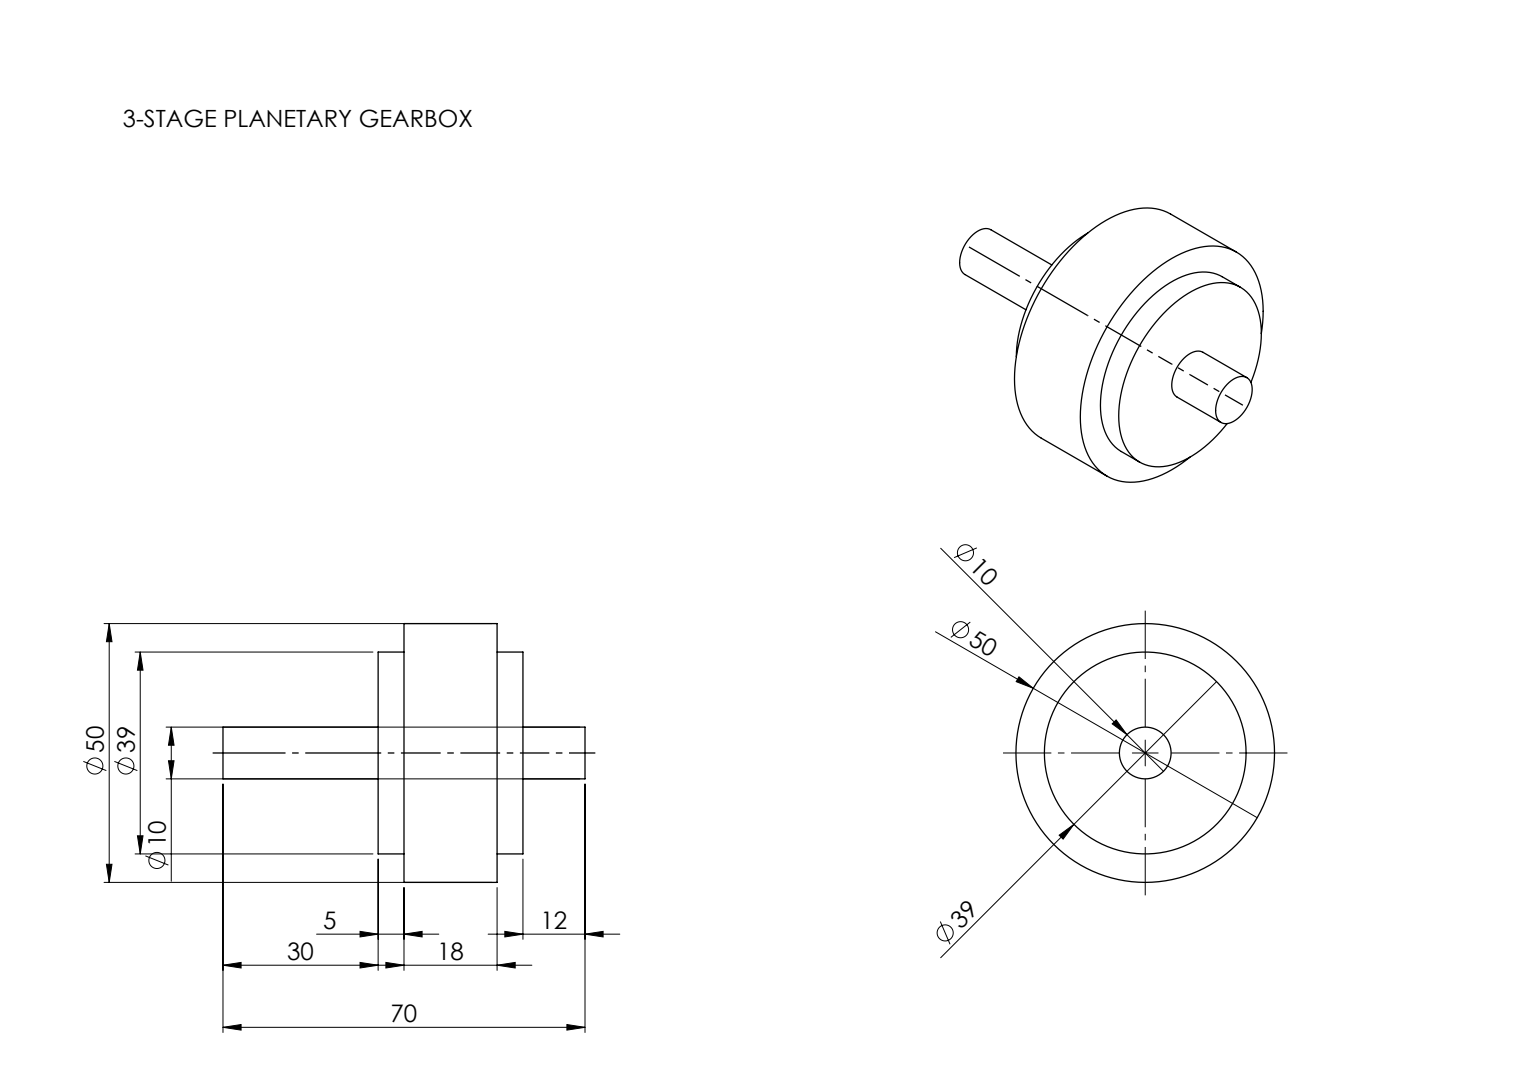
ISO-10303-21;
HEADER;
FILE_DESCRIPTION (('STEP AP214'),
    '1' );
FILE_NAME ('3-Stage Planetary Gearbox.step',
    '2026-10-05T20:22:16',
    ( '' ),
    ( '' ),
    'SwSTEP 2.0',
    'SolidWorks 2026',
    '' );
FILE_SCHEMA (( 'AUTOMOTIVE_DESIGN' ));
ENDSEC;

DATA;
#54=ORIENTED_EDGE ( 'NONE', *, *, #3388, .T. ) ;
#68=DIRECTION ( 'NONE',  ( 0.000000000000000000, 0.000000000000000000, 1.000000000000000000 ) ) ;
#87=DIRECTION ( 'NONE',  ( 0.000000000000000000, 0.000000000000000000, 1.000000000000000000 ) ) ;
#103=DIRECTION ( 'NONE',  ( 0.000000000000000000, 0.000000000000000000, 1.000000000000000000 ) ) ;
#119=ORIENTED_EDGE ( 'NONE', *, *, #7483, .T. ) ;
#126=ORIENTED_EDGE ( 'NONE', *, *, #14248, .F. ) ;
#235=EDGE_LOOP ( 'NONE', ( #13574, #321, #10866, #12718 ) ) ;
#261=CIRCLE ( 'NONE', #1953, 5.000000000000007994 ) ;
#301=CIRCLE ( 'NONE', #9619, 24.99999999999999645 ) ;
#313=VERTEX_POINT ( 'NONE', #2399 ) ;
#321=ORIENTED_EDGE ( 'NONE', *, *, #1465, .F. ) ;
#334=LINE ( 'NONE', #11212, #17228 ) ;
#345=EDGE_CURVE ( 'NONE', #10903, #313, #5234, .T. ) ;
#350=CARTESIAN_POINT ( 'NONE',  ( -50.00000000000000000, 171.6227766016838245, 24.99999999999999289 ) ) ;
#366=DIRECTION ( 'NONE',  ( -1.000000000000000000, -0.000000000000000000, -0.000000000000000000 ) ) ;
#432=AXIS2_PLACEMENT_3D ( 'NONE', #5586, #6655, #5500 ) ;
#446=EDGE_CURVE ( 'NONE', #9960, #12327, #12060, .T. ) ;
#485=CARTESIAN_POINT ( 'NONE',  ( -50.00000000000000000, 171.6227766016838245, 0.000000000000000000 ) ) ;
#508=DIRECTION ( 'NONE',  ( -1.000000000000000000, -0.000000000000000000, -0.000000000000000000 ) ) ;
#534=SURFACE_STYLE_USAGE ( .BOTH. , #5674 ) ;
#556=AXIS2_PLACEMENT_3D ( 'NONE', #15496, #7518, #2210 ) ;
#603=FACE_OUTER_BOUND ( 'NONE', #10174, .T. ) ;
#654=DIRECTION ( 'NONE',  ( -1.000000000000000000, 0.000000000000000000, 0.000000000000000000 ) ) ;
#713=VERTEX_POINT ( 'NONE', #3894 ) ;
#714=DIRECTION ( 'NONE',  ( 0.000000000000000000, 0.000000000000000000, -1.000000000000000000 ) ) ;
#771=FACE_BOUND ( 'NONE', #1719, .T. ) ;
#791=DIRECTION ( 'NONE',  ( -1.000000000000000000, 0.000000000000000000, 0.000000000000000000 ) ) ;
#836=CIRCLE ( 'NONE', #4239, 5.000000000000007994 ) ;
#866=AXIS2_PLACEMENT_3D ( 'NONE', #16436, #16167, #6863 ) ;
#886=ORIENTED_EDGE ( 'NONE', *, *, #9910, .T. ) ;
#990=CARTESIAN_POINT ( 'NONE',  ( -73.00000000000001421, 171.6227766016838245, 0.000000000000000000 ) ) ;
#1086=CARTESIAN_POINT ( 'NONE',  ( -73.00000000000001421, 171.6227766016838245, -5.000000000000007994 ) ) ;
#1147=CIRCLE ( 'NONE', #866, 24.99999999999999645 ) ;
#1200=DIRECTION ( 'NONE',  ( 0.000000000000000000, 0.000000000000000000, -1.000000000000000000 ) ) ;
#1235=FACE_OUTER_BOUND ( 'NONE', #1413, .T. ) ;
#1244=VECTOR ( 'NONE', #791, 1000.000000000000000 ) ;
#1354=DIRECTION ( 'NONE',  ( 0.000000000000000000, 0.000000000000000000, 1.000000000000000000 ) ) ;
#1360=ORIENTED_EDGE ( 'NONE', *, *, #6788, .T. ) ;
#1413=EDGE_LOOP ( 'NONE', ( #9423, #8176 ) ) ;
#1434=CIRCLE ( 'NONE', #13308, 5.000000000000007994 ) ;
#1465=EDGE_CURVE ( 'NONE', #10429, #16699, #5929, .T. ) ;
#1478=CARTESIAN_POINT ( 'NONE',  ( -33.00000000000000711, 171.6227766016838245, -5.000000000000007994 ) ) ;
#1490=CARTESIAN_POINT ( 'NONE',  ( -73.00000000000001421, 171.6227766016838245, 0.000000000000000000 ) ) ;
#1564=COLOUR_RGB ( '', 0.72549020, 0.75294118, 0.79215686) ;
#1569=CARTESIAN_POINT ( 'NONE',  ( -33.00000000000000711, 171.6227766016838245, 0.000000000000000000 ) ) ;
#1608=AXIS2_PLACEMENT_3D ( 'NONE', #16914, #3374, #714 ) ;
#1684=DIRECTION ( 'NONE',  ( -1.000000000000000000, 0.000000000000000000, 0.000000000000000000 ) ) ;
#1719=EDGE_LOOP ( 'NONE', ( #15688, #11199 ) ) ;
#1728=CARTESIAN_POINT ( 'NONE',  ( -33.00000000000000711, 171.6227766016838245, 0.000000000000000000 ) ) ;
#1778=ORIENTED_EDGE ( 'NONE', *, *, #14248, .T. ) ;
#1781=ORIENTED_EDGE ( 'NONE', *, *, #10186, .F. ) ;
#1805=DIRECTION ( 'NONE',  ( 0.000000000000000000, 0.000000000000000000, 1.000000000000000000 ) ) ;
#1843=PRESENTATION_STYLE_ASSIGNMENT (( #8568 ) ) ;
#1873=DIRECTION ( 'NONE',  ( -1.000000000000000000, 0.000000000000000000, 0.000000000000000000 ) ) ;
#1953=AXIS2_PLACEMENT_3D ( 'NONE', #16994, #6015, #10077 ) ;
#1978=DIRECTION ( 'NONE',  ( 1.000000000000000000, 0.000000000000000000, 0.000000000000000000 ) ) ;
#2008=CARTESIAN_POINT ( 'NONE',  ( -45.00000000000000711, 171.6227766016838245, -5.000000000000007994 ) ) ;
#2037=ORIENTED_EDGE ( 'NONE', *, *, #13494, .F. ) ;
#2046=UNCERTAINTY_MEASURE_WITH_UNIT (LENGTH_MEASURE( 1.000000000000000082E-05 ), #7499, 'distance_accuracy_value', 'NONE');
#2058=EDGE_LOOP ( 'NONE', ( #1778, #886 ) ) ;
#2072=ORIENTED_EDGE ( 'NONE', *, *, #8190, .F. ) ;
#2184=ORIENTED_EDGE ( 'NONE', *, *, #10068, .T. ) ;
#2188=FILL_AREA_STYLE ('',( #5926 ) ) ;
#2200=ADVANCED_FACE ( 'NONE', ( #13212 ), #4020, .T. ) ;
#2210=DIRECTION ( 'NONE',  ( 0.000000000000000000, 0.000000000000000000, -1.000000000000000000 ) ) ;
#2240=DIRECTION ( 'NONE',  ( -1.000000000000000000, 0.000000000000000000, 0.000000000000000000 ) ) ;
#2303=EDGE_CURVE ( 'NONE', #11799, #16546, #836, .T. ) ;
#2322=ORIENTED_EDGE ( 'NONE', *, *, #9701, .T. ) ;
#2362=SHAPE_REPRESENTATION_RELATIONSHIP ( 'NONE' , 'NONE' ,  #12790, #14383 ) ;
#2396=ADVANCED_FACE ( 'NONE', ( #12669 ), #3284, .T. ) ;
#2399=CARTESIAN_POINT ( 'NONE',  ( -68.00000000000000000, 171.6227766016838245, 19.49999999999998934 ) ) ;
#2467=PLANE ( 'NONE',  #11306 ) ;
#2489=ORIENTED_EDGE ( 'NONE', *, *, #8581, .F. ) ;
#2552=( NAMED_UNIT ( * ) PLANE_ANGLE_UNIT ( ) SI_UNIT ( $, .RADIAN. ) );
#2557=CIRCLE ( 'NONE', #16121, 19.49999999999998934 ) ;
#2567=ADVANCED_FACE ( 'NONE', ( #1235 ), #12129, .F. ) ;
#2626=CARTESIAN_POINT ( 'NONE',  ( -50.00000000000000000, 171.6227766016838245, -2.602085213965210642E-15 ) ) ;
#2685=DIRECTION ( 'NONE',  ( 1.000000000000000000, 0.000000000000000000, 0.000000000000000000 ) ) ;
#2730=DIRECTION ( 'NONE',  ( -1.000000000000000000, 0.000000000000000000, 0.000000000000000000 ) ) ;
#2731=CARTESIAN_POINT ( 'NONE',  ( -45.00000000000000711, 171.6227766016838245, -19.49999999999998224 ) ) ;
#2758=ORIENTED_EDGE ( 'NONE', *, *, #12197, .T. ) ;
#2824=ORIENTED_EDGE ( 'NONE', *, *, #12535, .F. ) ;
#2829=AXIS2_PLACEMENT_3D ( 'NONE', #6553, #17522, #5406 ) ;
#2961=ORIENTED_EDGE ( 'NONE', *, *, #9910, .F. ) ;
#3035=EDGE_LOOP ( 'NONE', ( #12238, #2184 ) ) ;
#3129=VERTEX_POINT ( 'NONE', #2008 ) ;
#3158=CIRCLE ( 'NONE', #9935, 19.49999999999998934 ) ;
#3169=DIRECTION ( 'NONE',  ( -1.000000000000000000, -0.000000000000000000, -0.000000000000000000 ) ) ;
#3187=( NAMED_UNIT ( * ) SI_UNIT ( $, .STERADIAN. ) SOLID_ANGLE_UNIT ( ) );
#3222=DIRECTION ( 'NONE',  ( 0.000000000000000000, 0.000000000000000000, 1.000000000000000000 ) ) ;
#3247=CYLINDRICAL_SURFACE ( 'NONE', #14920, 19.49999999999998224 ) ;
#3271=FILL_AREA_STYLE_COLOUR ( '', #1564 ) ;
#3284=PLANE ( 'NONE',  #17232 ) ;
#3288=FACE_OUTER_BOUND ( 'NONE', #16913, .T. ) ;
#3317=DIRECTION ( 'NONE',  ( 1.000000000000000000, 0.000000000000000000, 0.000000000000000000 ) ) ;
#3332=PRODUCT_DEFINITION_FORMATION_WITH_SPECIFIED_SOURCE ( 'ANY', '', #8417, .NOT_KNOWN. ) ;
#3365=CARTESIAN_POINT ( 'NONE',  ( -73.00000000000001421, 171.6227766016838245, 0.000000000000000000 ) ) ;
#3374=DIRECTION ( 'NONE',  ( 1.000000000000000000, -0.000000000000000000, -0.000000000000000000 ) ) ;
#3383=DIRECTION ( 'NONE',  ( -1.000000000000000000, -0.000000000000000000, -0.000000000000000000 ) ) ;
#3388=EDGE_CURVE ( 'NONE', #16699, #10429, #1147, .T. ) ;
#3457=ORIENTED_EDGE ( 'NONE', *, *, #4306, .T. ) ;
#3509=PLANE ( 'NONE',  #13524 ) ;
#3527=FACE_OUTER_BOUND ( 'NONE', #12622, .T. ) ;
#3582=AXIS2_PLACEMENT_3D ( 'NONE', #6896, #1684, #87 ) ;
#3583=AXIS2_PLACEMENT_3D ( 'NONE', #5482, #6893, #8222 ) ;
#3627=( GEOMETRIC_REPRESENTATION_CONTEXT ( 3 ) GLOBAL_UNCERTAINTY_ASSIGNED_CONTEXT ( ( #14095 ) ) GLOBAL_UNIT_ASSIGNED_CONTEXT ( ( #11921, #2552, #17326 ) ) REPRESENTATION_CONTEXT ( 'NONE', 'WORKASPACE' ) );
#3639=CIRCLE ( 'NONE', #13537, 19.49999999999998224 ) ;
#3654=AXIS2_PLACEMENT_3D ( 'NONE', #990, #2240, #13312 ) ;
#3668=ORIENTED_EDGE ( 'NONE', *, *, #4719, .T. ) ;
#3778=ORIENTED_EDGE ( 'NONE', *, *, #7387, .T. ) ;
#3827=AXIS2_PLACEMENT_3D ( 'NONE', #10507, #5024, #10415 ) ;
#3888=EDGE_LOOP ( 'NONE', ( #13542, #6426, #2824, #14641 ) ) ;
#3894=CARTESIAN_POINT ( 'NONE',  ( -45.00000000000000711, 171.6227766016838245, 5.000000000000007994 ) ) ;
#3933=CARTESIAN_POINT ( 'NONE',  ( -73.00000000000001421, 171.6227766016838245, -19.49999999999998934 ) ) ;
#4020=CYLINDRICAL_SURFACE ( 'NONE', #10166, 5.000000000000007994 ) ;
#4064=LINE ( 'NONE', #7952, #14405 ) ;
#4089=ORIENTED_EDGE ( 'NONE', *, *, #345, .F. ) ;
#4208=SHAPE_DEFINITION_REPRESENTATION ( #5739, #12790 ) ;
#4223=EDGE_CURVE ( 'NONE', #9434, #5867, #15502, .T. ) ;
#4239=AXIS2_PLACEMENT_3D ( 'NONE', #11072, #10987, #103 ) ;
#4306=EDGE_CURVE ( 'NONE', #11681, #4396, #3639, .T. ) ;
#4353=CYLINDRICAL_SURFACE ( 'NONE', #8087, 19.49999999999998224 ) ;
#4396=VERTEX_POINT ( 'NONE', #4661 ) ;
#4543=LINE ( 'NONE', #9929, #5507 ) ;
#4617=APPLICATION_CONTEXT ( 'automotive_design' ) ;
#4637=CARTESIAN_POINT ( 'NONE',  ( -138.7106781186547266, 171.6227766016838245, -2.602085213965210642E-15 ) ) ;
#4661=CARTESIAN_POINT ( 'NONE',  ( -50.00000000000000000, 171.6227766016838245, 19.49999999999998224 ) ) ;
#4719=EDGE_CURVE ( 'NONE', #5469, #10903, #11843, .T. ) ;
#4733=DIRECTION ( 'NONE',  ( 1.000000000000000000, 0.000000000000000000, 0.000000000000000000 ) ) ;
#4757=( GEOMETRIC_REPRESENTATION_CONTEXT ( 3 ) GLOBAL_UNCERTAINTY_ASSIGNED_CONTEXT ( ( #2046 ) ) GLOBAL_UNIT_ASSIGNED_CONTEXT ( ( #7499, #10066, #10160 ) ) REPRESENTATION_CONTEXT ( 'NONE', 'WORKASPACE' ) );
#4767=CIRCLE ( 'NONE', #15220, 19.49999999999998224 ) ;
#4779=CARTESIAN_POINT ( 'NONE',  ( -73.00000000000001421, 171.6227766016838245, 0.000000000000000000 ) ) ;
#4805=FACE_OUTER_BOUND ( 'NONE', #235, .T. ) ;
#4836=ORIENTED_EDGE ( 'NONE', *, *, #7483, .F. ) ;
#4859=EDGE_LOOP ( 'NONE', ( #12124, #5327, #2758, #14191 ) ) ;
#4915=AXIS2_PLACEMENT_3D ( 'NONE', #11281, #4733, #8802 ) ;
#5024=DIRECTION ( 'NONE',  ( 1.000000000000000000, 0.000000000000000000, 0.000000000000000000 ) ) ;
#5056=EDGE_LOOP ( 'NONE', ( #6270, #2037 ) ) ;
#5077=ORIENTED_EDGE ( 'NONE', *, *, #9244, .T. ) ;
#5138=DIRECTION ( 'NONE',  ( -1.000000000000000000, 0.000000000000000000, 0.000000000000000000 ) ) ;
#5158=DIRECTION ( 'NONE',  ( -1.000000000000000000, 0.000000000000000000, 0.000000000000000000 ) ) ;
#5173=ADVANCED_FACE ( 'NONE', ( #6711, #6345 ), #14415, .T. ) ;
#5234=LINE ( 'NONE', #10633, #16593 ) ;
#5316=ADVANCED_FACE ( 'NONE', ( #8375 ), #12367, .T. ) ;
#5327=ORIENTED_EDGE ( 'NONE', *, *, #345, .T. ) ;
#5406=DIRECTION ( 'NONE',  ( 0.000000000000000000, 0.000000000000000000, 1.000000000000000000 ) ) ;
#5414=CARTESIAN_POINT ( 'NONE',  ( -103.0000000000000142, 171.6227766016838245, -5.000000000000007994 ) ) ;
#5469=VERTEX_POINT ( 'NONE', #6416 ) ;
#5482=CARTESIAN_POINT ( 'NONE',  ( 0.000000000000000000, 0.000000000000000000, 0.000000000000000000 ) ) ;
#5500=DIRECTION ( 'NONE',  ( 0.000000000000000000, 0.000000000000000000, 1.000000000000000000 ) ) ;
#5507=VECTOR ( 'NONE', #5958, 1000.000000000000000 ) ;
#5562=DIRECTION ( 'NONE',  ( 0.000000000000000000, 0.000000000000000000, -1.000000000000000000 ) ) ;
#5586=CARTESIAN_POINT ( 'NONE',  ( -68.00000000000000000, 171.6227766016838245, 0.000000000000000000 ) ) ;
#5674=SURFACE_SIDE_STYLE ('',( #16656 ) ) ;
#5698=VECTOR ( 'NONE', #3317, 1000.000000000000000 ) ;
#5739=PRODUCT_DEFINITION_SHAPE ( 'NONE', 'NONE',  #10297 ) ;
#5813=ADVANCED_FACE ( 'NONE', ( #14203 ), #8534, .T. ) ;
#5833=CIRCLE ( 'NONE', #14034, 19.49999999999998224 ) ;
#5837=DIRECTION ( 'NONE',  ( 0.000000000000000000, 0.000000000000000000, -1.000000000000000000 ) ) ;
#5856=CARTESIAN_POINT ( 'NONE',  ( -45.00000000000000711, 171.6227766016838245, 0.000000000000000000 ) ) ;
#5867=VERTEX_POINT ( 'NONE', #1086 ) ;
#5872=AXIS2_PLACEMENT_3D ( 'NONE', #1569, #2730, #9622 ) ;
#5894=MECHANICAL_DESIGN_GEOMETRIC_PRESENTATION_REPRESENTATION('',(#13811),#3627);
#5926=FILL_AREA_STYLE_COLOUR ( '', #6743 ) ;
#5929=CIRCLE ( 'NONE', #556, 24.99999999999999645 ) ;
#5957=DIRECTION ( 'NONE',  ( -1.000000000000000000, 0.000000000000000000, 0.000000000000000000 ) ) ;
#5958=DIRECTION ( 'NONE',  ( -1.000000000000000000, 0.000000000000000000, 0.000000000000000000 ) ) ;
#6015=DIRECTION ( 'NONE',  ( -1.000000000000000000, 0.000000000000000000, 0.000000000000000000 ) ) ;
#6025=FACE_OUTER_BOUND ( 'NONE', #4859, .T. ) ;
#6087=ORIENTED_EDGE ( 'NONE', *, *, #2303, .T. ) ;
#6187=DIRECTION ( 'NONE',  ( 0.000000000000000000, 0.000000000000000000, 1.000000000000000000 ) ) ;
#6205=ADVANCED_FACE ( 'NONE', ( #3288 ), #4353, .T. ) ;
#6270=ORIENTED_EDGE ( 'NONE', *, *, #4223, .F. ) ;
#6272=DIRECTION ( 'NONE',  ( 1.000000000000000000, -0.000000000000000000, -0.000000000000000000 ) ) ;
#6345=FACE_OUTER_BOUND ( 'NONE', #2058, .T. ) ;
#6380=CLOSED_SHELL ( 'NONE', ( #5813, #13369, #6205, #16486, #17351, #15245, #13690, #15493, #10124, #8032, #13534, #5173, #2567, #2200, #5316, #2396 ) ) ;
#6416=CARTESIAN_POINT ( 'NONE',  ( -73.00000000000001421, 171.6227766016838245, -19.49999999999998934 ) ) ;
#6426=ORIENTED_EDGE ( 'NONE', *, *, #17427, .T. ) ;
#6543=FACE_OUTER_BOUND ( 'NONE', #9128, .T. ) ;
#6553=CARTESIAN_POINT ( 'NONE',  ( -33.00000000000000711, 171.6227766016838245, 0.000000000000000000 ) ) ;
#6591=ORIENTED_EDGE ( 'NONE', *, *, #13494, .T. ) ;
#6655=DIRECTION ( 'NONE',  ( 1.000000000000000000, 0.000000000000000000, -0.000000000000000000 ) ) ;
#6656=DIRECTION ( 'NONE',  ( 1.000000000000000000, -0.000000000000000000, -0.000000000000000000 ) ) ;
#6711=FACE_BOUND ( 'NONE', #9913, .T. ) ;
#6718=DIRECTION ( 'NONE',  ( -1.000000000000000000, 0.000000000000000000, 0.000000000000000000 ) ) ;
#6720=DIRECTION ( 'NONE',  ( 1.000000000000000000, 0.000000000000000000, 0.000000000000000000 ) ) ;
#6727=CARTESIAN_POINT ( 'NONE',  ( -33.00000000000000711, 171.6227766016838245, 5.000000000000007994 ) ) ;
#6743=COLOUR_RGB ( '', 0.72549020, 0.75294118, 0.79215686) ;
#6768=AXIS2_PLACEMENT_3D ( 'NONE', #4779, #6272, #15573 ) ;
#6788=EDGE_CURVE ( 'NONE', #9434, #14250, #13005, .T. ) ;
#6863=DIRECTION ( 'NONE',  ( 0.000000000000000000, 0.000000000000000000, -1.000000000000000000 ) ) ;
#6893=DIRECTION ( 'NONE',  ( 0.000000000000000000, 0.000000000000000000, 1.000000000000000000 ) ) ;
#6896=CARTESIAN_POINT ( 'NONE',  ( -103.0000000000000142, 171.6227766016838245, 0.000000000000000000 ) ) ;
#6905=ORIENTED_EDGE ( 'NONE', *, *, #10186, .T. ) ;
#6979=ORIENTED_EDGE ( 'NONE', *, *, #4719, .F. ) ;
#7030=AXIS2_PLACEMENT_3D ( 'NONE', #8289, #8473, #68 ) ;
#7106=DIRECTION ( 'NONE',  ( 0.000000000000000000, 0.000000000000000000, -1.000000000000000000 ) ) ;
#7119=EDGE_CURVE ( 'NONE', #713, #3129, #11994, .T. ) ;
#7142=CARTESIAN_POINT ( 'NONE',  ( -33.00000000000000711, 171.6227766016838245, 0.000000000000000000 ) ) ;
#7165=DIRECTION ( 'NONE',  ( 1.000000000000000000, 0.000000000000000000, 0.000000000000000000 ) ) ;
#7186=DIRECTION ( 'NONE',  ( 1.000000000000000000, 0.000000000000000000, 0.000000000000000000 ) ) ;
#7255=( LENGTH_UNIT ( ) NAMED_UNIT ( * ) SI_UNIT ( .MILLI., .METRE. ) );
#7327=CIRCLE ( 'NONE', #14121, 19.49999999999998224 ) ;
#7335=EDGE_CURVE ( 'NONE', #10429, #12327, #8425, .T. ) ;
#7382=DIRECTION ( 'NONE',  ( 0.000000000000000000, 0.000000000000000000, -1.000000000000000000 ) ) ;
#7387=EDGE_CURVE ( 'NONE', #16546, #713, #4543, .T. ) ;
#7389=DIRECTION ( 'NONE',  ( -1.000000000000000000, 0.000000000000000000, 0.000000000000000000 ) ) ;
#7422=ORIENTED_EDGE ( 'NONE', *, *, #12197, .F. ) ;
#7483=EDGE_CURVE ( 'NONE', #15075, #4396, #10099, .T. ) ;
#7485=DIRECTION ( 'NONE',  ( 0.000000000000000000, 0.000000000000000000, 1.000000000000000000 ) ) ;
#7499=( LENGTH_UNIT ( ) NAMED_UNIT ( * ) SI_UNIT ( .MILLI., .METRE. ) );
#7518=DIRECTION ( 'NONE',  ( -1.000000000000000000, -0.000000000000000000, -0.000000000000000000 ) ) ;
#7538=DIRECTION ( 'NONE',  ( 1.000000000000000000, 0.000000000000000000, 0.000000000000000000 ) ) ;
#7706=CARTESIAN_POINT ( 'NONE',  ( -138.7106781186547266, 171.6227766016838245, -2.602085213965210642E-15 ) ) ;
#7713=ORIENTED_EDGE ( 'NONE', *, *, #8581, .T. ) ;
#7724=EDGE_LOOP ( 'NONE', ( #10611, #7422 ) ) ;
#7762=DIRECTION ( 'NONE',  ( -1.000000000000000000, 0.000000000000000000, 0.000000000000000000 ) ) ;
#7872=CARTESIAN_POINT ( 'NONE',  ( -33.00000000000000711, 171.6227766016838245, -5.000000000000007994 ) ) ;
#7910=EDGE_CURVE ( 'NONE', #10903, #5469, #2557, .T. ) ;
#7952=CARTESIAN_POINT ( 'NONE',  ( -33.00000000000000711, 171.6227766016838245, -5.000000000000007994 ) ) ;
#7993=ORIENTED_EDGE ( 'NONE', *, *, #1465, .T. ) ;
#8032=ADVANCED_FACE ( 'NONE', ( #10424, #6543 ), #2467, .T. ) ;
#8058=FACE_BOUND ( 'NONE', #7724, .T. ) ;
#8087=AXIS2_PLACEMENT_3D ( 'NONE', #5856, #366, #11156 ) ;
#8097=DIRECTION ( 'NONE',  ( 0.000000000000000000, 0.000000000000000000, -1.000000000000000000 ) ) ;
#8128=ORIENTED_EDGE ( 'NONE', *, *, #446, .T. ) ;
#8176=ORIENTED_EDGE ( 'NONE', *, *, #2303, .F. ) ;
#8190=EDGE_CURVE ( 'NONE', #3129, #713, #1434, .T. ) ;
#8222=DIRECTION ( 'NONE',  ( 1.000000000000000000, 0.000000000000000000, 0.000000000000000000 ) ) ;
#8232=CARTESIAN_POINT ( 'NONE',  ( -45.00000000000000711, 171.6227766016838245, 0.000000000000000000 ) ) ;
#8289=CARTESIAN_POINT ( 'NONE',  ( -73.00000000000001421, 171.6227766016838245, 0.000000000000000000 ) ) ;
#8375=FACE_OUTER_BOUND ( 'NONE', #12203, .T. ) ;
#8378=AXIS2_PLACEMENT_3D ( 'NONE', #14880, #9561, #13729 ) ;
#8381=FACE_OUTER_BOUND ( 'NONE', #9058, .T. ) ;
#8404=ORIENTED_EDGE ( 'NONE', *, *, #9479, .T. ) ;
#8417=PRODUCT ( '3-Stage Planetary Gearbox', '3-Stage Planetary Gearbox', '', ( #9766 ) ) ;
#8425=LINE ( 'NONE', #13844, #14259 ) ;
#8432=CARTESIAN_POINT ( 'NONE',  ( -45.00000000000000711, 171.6227766016838245, 19.49999999999998224 ) ) ;
#8441=FACE_OUTER_BOUND ( 'NONE', #16137, .T. ) ;
#8473=DIRECTION ( 'NONE',  ( -1.000000000000000000, 0.000000000000000000, 0.000000000000000000 ) ) ;
#8534=CYLINDRICAL_SURFACE ( 'NONE', #13173, 5.000000000000007994 ) ;
#8568=SURFACE_STYLE_USAGE ( .BOTH. , #11319 ) ;
#8581=EDGE_CURVE ( 'NONE', #12327, #9960, #301, .T. ) ;
#8802=DIRECTION ( 'NONE',  ( 0.000000000000000000, 0.000000000000000000, -1.000000000000000000 ) ) ;
#8850=DIRECTION ( 'NONE',  ( 0.000000000000000000, 0.000000000000000000, 1.000000000000000000 ) ) ;
#9005=CARTESIAN_POINT ( 'NONE',  ( -33.00000000000000711, 171.6227766016838245, 5.000000000000007994 ) ) ;
#9058=EDGE_LOOP ( 'NONE', ( #5077, #6905, #10220, #11040 ) ) ;
#9128=EDGE_LOOP ( 'NONE', ( #3668, #12856 ) ) ;
#9244=EDGE_CURVE ( 'NONE', #16546, #11799, #9638, .T. ) ;
#9286=LINE ( 'NONE', #7872, #11240 ) ;
#9307=EDGE_CURVE ( 'NONE', #16699, #9960, #15347, .T. ) ;
#9317=LINE ( 'NONE', #3933, #12764 ) ;
#9366=DIRECTION ( 'NONE',  ( -1.000000000000000000, 0.000000000000000000, 0.000000000000000000 ) ) ;
#9423=ORIENTED_EDGE ( 'NONE', *, *, #9244, .F. ) ;
#9434=VERTEX_POINT ( 'NONE', #12866 ) ;
#9462=( GEOMETRIC_REPRESENTATION_CONTEXT ( 3 ) GLOBAL_UNCERTAINTY_ASSIGNED_CONTEXT ( ( #10564 ) ) GLOBAL_UNIT_ASSIGNED_CONTEXT ( ( #7255, #12487, #3187 ) ) REPRESENTATION_CONTEXT ( 'NONE', 'WORKASPACE' ) );
#9473=AXIS2_PLACEMENT_3D ( 'NONE', #7142, #13794, #12541 ) ;
#9479=EDGE_CURVE ( 'NONE', #5469, #17135, #9317, .T. ) ;
#9509=CARTESIAN_POINT ( 'NONE',  ( -50.00000000000000000, 171.6227766016838245, -2.602085213965210642E-15 ) ) ;
#9561=DIRECTION ( 'NONE',  ( 1.000000000000000000, 0.000000000000000000, 0.000000000000000000 ) ) ;
#9619=AXIS2_PLACEMENT_3D ( 'NONE', #2626, #14662, #8097 ) ;
#9622=DIRECTION ( 'NONE',  ( 0.000000000000000000, 0.000000000000000000, 1.000000000000000000 ) ) ;
#9638=CIRCLE ( 'NONE', #12484, 5.000000000000007994 ) ;
#9701=EDGE_CURVE ( 'NONE', #17135, #313, #3158, .T. ) ;
#9745=DIRECTION ( 'NONE',  ( 0.000000000000000000, 0.000000000000000000, 1.000000000000000000 ) ) ;
#9766=PRODUCT_CONTEXT ( 'NONE', #4617, 'mechanical' ) ;
#9842=ORIENTED_EDGE ( 'NONE', *, *, #10337, .F. ) ;
#9898=VERTEX_POINT ( 'NONE', #5414 ) ;
#9910=EDGE_CURVE ( 'NONE', #10212, #15075, #7327, .T. ) ;
#9913=EDGE_LOOP ( 'NONE', ( #15725, #2072 ) ) ;
#9929=CARTESIAN_POINT ( 'NONE',  ( -33.00000000000000711, 171.6227766016838245, 5.000000000000007994 ) ) ;
#9935=AXIS2_PLACEMENT_3D ( 'NONE', #13842, #5957, #9745 ) ;
#9960=VERTEX_POINT ( 'NONE', #350 ) ;
#10051=CARTESIAN_POINT ( 'NONE',  ( -45.00000000000000711, 171.6227766016838245, 0.000000000000000000 ) ) ;
#10066=( NAMED_UNIT ( * ) PLANE_ANGLE_UNIT ( ) SI_UNIT ( $, .RADIAN. ) );
#10068=EDGE_CURVE ( 'NONE', #9898, #14250, #261, .T. ) ;
#10077=DIRECTION ( 'NONE',  ( 0.000000000000000000, 0.000000000000000000, 1.000000000000000000 ) ) ;
#10098=AXIS2_PLACEMENT_3D ( 'NONE', #1490, #6718, #12277 ) ;
#10099=LINE ( 'NONE', #15506, #16531 ) ;
#10124=ADVANCED_FACE ( 'NONE', ( #3527 ), #16904, .T. ) ;
#10136=CARTESIAN_POINT ( 'NONE',  ( -68.00000000000000000, 171.6227766016838245, -19.49999999999998934 ) ) ;
#10160=( NAMED_UNIT ( * ) SI_UNIT ( $, .STERADIAN. ) SOLID_ANGLE_UNIT ( ) );
#10166=AXIS2_PLACEMENT_3D ( 'NONE', #13573, #5158, #1354 ) ;
#10174=EDGE_LOOP ( 'NONE', ( #9842, #126, #119, #10975 ) ) ;
#10180=CYLINDRICAL_SURFACE ( 'NONE', #1608, 19.49999999999998934 ) ;
#10186=EDGE_CURVE ( 'NONE', #11799, #3129, #4064, .T. ) ;
#10212=VERTEX_POINT ( 'NONE', #2731 ) ;
#10220=ORIENTED_EDGE ( 'NONE', *, *, #8190, .T. ) ;
#10272=CYLINDRICAL_SURFACE ( 'NONE', #12423, 24.99999999999999645 ) ;
#10297=PRODUCT_DEFINITION ( 'UNKNOWN', '', #3332, #11026 ) ;
#10337=EDGE_CURVE ( 'NONE', #10212, #11681, #334, .T. ) ;
#10381=CIRCLE ( 'NONE', #10098, 5.000000000000007994 ) ;
#10415=DIRECTION ( 'NONE',  ( 0.000000000000000000, 0.000000000000000000, -1.000000000000000000 ) ) ;
#10424=FACE_BOUND ( 'NONE', #5056, .T. ) ;
#10429=VERTEX_POINT ( 'NONE', #16459 ) ;
#10456=DIRECTION ( 'NONE',  ( 0.000000000000000000, 0.000000000000000000, -1.000000000000000000 ) ) ;
#10507=CARTESIAN_POINT ( 'NONE',  ( -45.00000000000000711, 171.6227766016838245, 0.000000000000000000 ) ) ;
#10564=UNCERTAINTY_MEASURE_WITH_UNIT (LENGTH_MEASURE( 1.000000000000000082E-05 ), #7255, 'distance_accuracy_value', 'NONE');
#10611=ORIENTED_EDGE ( 'NONE', *, *, #9701, .F. ) ;
#10633=CARTESIAN_POINT ( 'NONE',  ( -73.00000000000001421, 171.6227766016838245, 19.49999999999998934 ) ) ;
#10866=ORIENTED_EDGE ( 'NONE', *, *, #7335, .T. ) ;
#10903=VERTEX_POINT ( 'NONE', #11080 ) ;
#10905=AXIS2_PLACEMENT_3D ( 'NONE', #13754, #16239, #16422 ) ;
#10975=ORIENTED_EDGE ( 'NONE', *, *, #11916, .T. ) ;
#10987=DIRECTION ( 'NONE',  ( -1.000000000000000000, 0.000000000000000000, 0.000000000000000000 ) ) ;
#11021=DIRECTION ( 'NONE',  ( 1.000000000000000000, 0.000000000000000000, 0.000000000000000000 ) ) ;
#11026=PRODUCT_DEFINITION_CONTEXT ( 'detailed design', #14555, 'design' ) ;
#11040=ORIENTED_EDGE ( 'NONE', *, *, #7387, .F. ) ;
#11063=FILL_AREA_STYLE ('',( #3271 ) ) ;
#11072=CARTESIAN_POINT ( 'NONE',  ( -33.00000000000000711, 171.6227766016838245, 0.000000000000000000 ) ) ;
#11080=CARTESIAN_POINT ( 'NONE',  ( -73.00000000000001421, 171.6227766016838245, 19.49999999999998934 ) ) ;
#11148=MANIFOLD_SOLID_BREP ( 'Boss-Extrude4', #6380 ) ;
#11156=DIRECTION ( 'NONE',  ( 0.000000000000000000, 0.000000000000000000, 1.000000000000000000 ) ) ;
#11185=CARTESIAN_POINT ( 'NONE',  ( -138.7106781186547266, 171.6227766016838245, 24.99999999999999289 ) ) ;
#11199=ORIENTED_EDGE ( 'NONE', *, *, #4306, .F. ) ;
#11212=CARTESIAN_POINT ( 'NONE',  ( -45.00000000000000711, 171.6227766016838245, -19.49999999999998224 ) ) ;
#11240=VECTOR ( 'NONE', #5138, 1000.000000000000000 ) ;
#11281=CARTESIAN_POINT ( 'NONE',  ( -45.00000000000000711, 171.6227766016838245, 0.000000000000000000 ) ) ;
#11306=AXIS2_PLACEMENT_3D ( 'NONE', #17156, #7762, #12918 ) ;
#11319=SURFACE_SIDE_STYLE ('',( #15304 ) ) ;
#11417=CARTESIAN_POINT ( 'NONE',  ( -103.0000000000000142, 171.6227766016838245, 0.000000000000000000 ) ) ;
#11681=VERTEX_POINT ( 'NONE', #17505 ) ;
#11799=VERTEX_POINT ( 'NONE', #1478 ) ;
#11843=CIRCLE ( 'NONE', #3654, 19.49999999999998934 ) ;
#11916=EDGE_CURVE ( 'NONE', #4396, #11681, #5833, .T. ) ;
#11921=( LENGTH_UNIT ( ) NAMED_UNIT ( * ) SI_UNIT ( .MILLI., .METRE. ) );
#11980=ORIENTED_EDGE ( 'NONE', *, *, #10337, .T. ) ;
#11994=CIRCLE ( 'NONE', #4915, 5.000000000000007994 ) ;
#12002=EDGE_LOOP ( 'NONE', ( #7713, #8128 ) ) ;
#12060=CIRCLE ( 'NONE', #8378, 24.99999999999999645 ) ;
#12124=ORIENTED_EDGE ( 'NONE', *, *, #7910, .F. ) ;
#12129=PLANE ( 'NONE',  #2829 ) ;
#12197=EDGE_CURVE ( 'NONE', #313, #17135, #13750, .T. ) ;
#12203=EDGE_LOOP ( 'NONE', ( #12406, #6591, #1360, #14687 ) ) ;
#12238=ORIENTED_EDGE ( 'NONE', *, *, #12535, .T. ) ;
#12277=DIRECTION ( 'NONE',  ( 0.000000000000000000, 0.000000000000000000, 1.000000000000000000 ) ) ;
#12327=VERTEX_POINT ( 'NONE', #16127 ) ;
#12367=CYLINDRICAL_SURFACE ( 'NONE', #9473, 5.000000000000007994 ) ;
#12406=ORIENTED_EDGE ( 'NONE', *, *, #17427, .F. ) ;
#12423=AXIS2_PLACEMENT_3D ( 'NONE', #7706, #7538, #10456 ) ;
#12466=CYLINDRICAL_SURFACE ( 'NONE', #5872, 5.000000000000007994 ) ;
#12484=AXIS2_PLACEMENT_3D ( 'NONE', #13771, #7389, #3222 ) ;
#12487=( NAMED_UNIT ( * ) PLANE_ANGLE_UNIT ( ) SI_UNIT ( $, .RADIAN. ) );
#12493=ORIENTED_EDGE ( 'NONE', *, *, #7119, .T. ) ;
#12535=EDGE_CURVE ( 'NONE', #14250, #9898, #13767, .T. ) ;
#12541=DIRECTION ( 'NONE',  ( 0.000000000000000000, 0.000000000000000000, 1.000000000000000000 ) ) ;
#12622=EDGE_LOOP ( 'NONE', ( #4089, #6979, #8404, #2322 ) ) ;
#12669=FACE_OUTER_BOUND ( 'NONE', #3035, .T. ) ;
#12718=ORIENTED_EDGE ( 'NONE', *, *, #446, .F. ) ;
#12764=VECTOR ( 'NONE', #13395, 1000.000000000000000 ) ;
#12790=SHAPE_REPRESENTATION ( '3-Stage Planetary Gearbox', ( #3583 ), #4757 ) ;
#12856=ORIENTED_EDGE ( 'NONE', *, *, #7910, .T. ) ;
#12866=CARTESIAN_POINT ( 'NONE',  ( -73.00000000000001421, 171.6227766016838245, 5.000000000000007994 ) ) ;
#12896=FACE_OUTER_BOUND ( 'NONE', #12002, .T. ) ;
#12918=DIRECTION ( 'NONE',  ( 0.000000000000000000, 0.000000000000000000, 1.000000000000000000 ) ) ;
#12941=AXIS2_PLACEMENT_3D ( 'NONE', #4637, #1978, #7382 ) ;
#13005=LINE ( 'NONE', #9005, #1244 ) ;
#13076=EDGE_LOOP ( 'NONE', ( #7993, #54 ) ) ;
#13173=AXIS2_PLACEMENT_3D ( 'NONE', #1728, #654, #1805 ) ;
#13178=DIRECTION ( 'NONE',  ( -1.000000000000000000, 0.000000000000000000, 0.000000000000000000 ) ) ;
#13212=FACE_OUTER_BOUND ( 'NONE', #14487, .T. ) ;
#13308=AXIS2_PLACEMENT_3D ( 'NONE', #14773, #6720, #5562 ) ;
#13312=DIRECTION ( 'NONE',  ( 0.000000000000000000, 0.000000000000000000, 1.000000000000000000 ) ) ;
#13369=ADVANCED_FACE ( 'NONE', ( #8381 ), #12466, .T. ) ;
#13395=DIRECTION ( 'NONE',  ( 1.000000000000000000, -0.000000000000000000, -0.000000000000000000 ) ) ;
#13445=MECHANICAL_DESIGN_GEOMETRIC_PRESENTATION_REPRESENTATION('',(#14006),#9462);
#13469=PLANE ( 'NONE',  #432 ) ;
#13494=EDGE_CURVE ( 'NONE', #5867, #9434, #10381, .T. ) ;
#13524=AXIS2_PLACEMENT_3D ( 'NONE', #9509, #11021, #1200 ) ;
#13534=ADVANCED_FACE ( 'NONE', ( #603 ), #3247, .T. ) ;
#13537=AXIS2_PLACEMENT_3D ( 'NONE', #13966, #16795, #15366 ) ;
#13542=ORIENTED_EDGE ( 'NONE', *, *, #4223, .T. ) ;
#13573=CARTESIAN_POINT ( 'NONE',  ( -33.00000000000000711, 171.6227766016838245, 0.000000000000000000 ) ) ;
#13574=ORIENTED_EDGE ( 'NONE', *, *, #9307, .F. ) ;
#13645=FACE_OUTER_BOUND ( 'NONE', #13076, .T. ) ;
#13690=ADVANCED_FACE ( 'NONE', ( #771, #12896 ), #3509, .T. ) ;
#13729=DIRECTION ( 'NONE',  ( 0.000000000000000000, 0.000000000000000000, -1.000000000000000000 ) ) ;
#13750=CIRCLE ( 'NONE', #10905, 19.49999999999998934 ) ;
#13754=CARTESIAN_POINT ( 'NONE',  ( -68.00000000000000000, 171.6227766016838245, 0.000000000000000000 ) ) ;
#13767=CIRCLE ( 'NONE', #3582, 5.000000000000007994 ) ;
#13771=CARTESIAN_POINT ( 'NONE',  ( -33.00000000000000711, 171.6227766016838245, 0.000000000000000000 ) ) ;
#13794=DIRECTION ( 'NONE',  ( -1.000000000000000000, 0.000000000000000000, 0.000000000000000000 ) ) ;
#13811=STYLED_ITEM ( 'NONE', ( #1843 ), #14383 ) ;
#13842=CARTESIAN_POINT ( 'NONE',  ( -68.00000000000000000, 171.6227766016838245, 0.000000000000000000 ) ) ;
#13844=CARTESIAN_POINT ( 'NONE',  ( -138.7106781186547266, 171.6227766016838245, -25.00000000000000000 ) ) ;
#13966=CARTESIAN_POINT ( 'NONE',  ( -50.00000000000000000, 171.6227766016838245, 0.000000000000000000 ) ) ;
#14006=STYLED_ITEM ( 'NONE', ( #16477 ), #11148 ) ;
#14034=AXIS2_PLACEMENT_3D ( 'NONE', #485, #14290, #15445 ) ;
#14095=UNCERTAINTY_MEASURE_WITH_UNIT (LENGTH_MEASURE( 1.000000000000000082E-05 ), #11921, 'distance_accuracy_value', 'NONE');
#14121=AXIS2_PLACEMENT_3D ( 'NONE', #8232, #7165, #5837 ) ;
#14191=ORIENTED_EDGE ( 'NONE', *, *, #9479, .F. ) ;
#14203=FACE_OUTER_BOUND ( 'NONE', #3888, .T. ) ;
#14248=EDGE_CURVE ( 'NONE', #15075, #10212, #4767, .T. ) ;
#14250=VERTEX_POINT ( 'NONE', #17015 ) ;
#14259=VECTOR ( 'NONE', #2685, 1000.000000000000000 ) ;
#14290=DIRECTION ( 'NONE',  ( 1.000000000000000000, 0.000000000000000000, 0.000000000000000000 ) ) ;
#14383=ADVANCED_BREP_SHAPE_REPRESENTATION ( '', ( #11148, #3583 ), #4757 ) ;
#14405=VECTOR ( 'NONE', #9366, 1000.000000000000000 ) ;
#14415=PLANE ( 'NONE',  #3827 ) ;
#14452=ORIENTED_EDGE ( 'NONE', *, *, #3388, .F. ) ;
#14487=EDGE_LOOP ( 'NONE', ( #1781, #6087, #3778, #12493 ) ) ;
#14555=APPLICATION_CONTEXT ( 'automotive_design' ) ;
#14641=ORIENTED_EDGE ( 'NONE', *, *, #6788, .F. ) ;
#14662=DIRECTION ( 'NONE',  ( 1.000000000000000000, 0.000000000000000000, 0.000000000000000000 ) ) ;
#14687=ORIENTED_EDGE ( 'NONE', *, *, #10068, .F. ) ;
#14738=ORIENTED_EDGE ( 'NONE', *, *, #9307, .T. ) ;
#14773=CARTESIAN_POINT ( 'NONE',  ( -45.00000000000000711, 171.6227766016838245, 0.000000000000000000 ) ) ;
#14880=CARTESIAN_POINT ( 'NONE',  ( -50.00000000000000000, 171.6227766016838245, -2.602085213965210642E-15 ) ) ;
#14920=AXIS2_PLACEMENT_3D ( 'NONE', #10051, #508, #7485 ) ;
#15075=VERTEX_POINT ( 'NONE', #8432 ) ;
#15209=CARTESIAN_POINT ( 'NONE',  ( -68.00000000000000000, 171.6227766016838245, 24.99999999999999289 ) ) ;
#15220=AXIS2_PLACEMENT_3D ( 'NONE', #16763, #7186, #7106 ) ;
#15245=ADVANCED_FACE ( 'NONE', ( #4805 ), #10272, .T. ) ;
#15304=SURFACE_STYLE_FILL_AREA ( #2188 ) ;
#15347=LINE ( 'NONE', #11185, #5698 ) ;
#15366=DIRECTION ( 'NONE',  ( 0.000000000000000000, 0.000000000000000000, -1.000000000000000000 ) ) ;
#15445=DIRECTION ( 'NONE',  ( 0.000000000000000000, 0.000000000000000000, -1.000000000000000000 ) ) ;
#15493=ADVANCED_FACE ( 'NONE', ( #8058, #13645 ), #13469, .F. ) ;
#15496=CARTESIAN_POINT ( 'NONE',  ( -68.00000000000000000, 171.6227766016838245, -2.602085213965210642E-15 ) ) ;
#15502=CIRCLE ( 'NONE', #7030, 5.000000000000007994 ) ;
#15506=CARTESIAN_POINT ( 'NONE',  ( -45.00000000000000711, 171.6227766016838245, 19.49999999999998224 ) ) ;
#15573=DIRECTION ( 'NONE',  ( 0.000000000000000000, 0.000000000000000000, -1.000000000000000000 ) ) ;
#15688=ORIENTED_EDGE ( 'NONE', *, *, #11916, .F. ) ;
#15725=ORIENTED_EDGE ( 'NONE', *, *, #7119, .F. ) ;
#16121=AXIS2_PLACEMENT_3D ( 'NONE', #3365, #13178, #6187 ) ;
#16127=CARTESIAN_POINT ( 'NONE',  ( -50.00000000000000000, 171.6227766016838245, -25.00000000000000000 ) ) ;
#16137=EDGE_LOOP ( 'NONE', ( #14452, #14738, #2489, #17247 ) ) ;
#16167=DIRECTION ( 'NONE',  ( -1.000000000000000000, -0.000000000000000000, -0.000000000000000000 ) ) ;
#16239=DIRECTION ( 'NONE',  ( -1.000000000000000000, 0.000000000000000000, 0.000000000000000000 ) ) ;
#16422=DIRECTION ( 'NONE',  ( 0.000000000000000000, 0.000000000000000000, 1.000000000000000000 ) ) ;
#16436=CARTESIAN_POINT ( 'NONE',  ( -68.00000000000000000, 171.6227766016838245, -2.602085213965210642E-15 ) ) ;
#16459=CARTESIAN_POINT ( 'NONE',  ( -68.00000000000000000, 171.6227766016838245, -25.00000000000000000 ) ) ;
#16477=PRESENTATION_STYLE_ASSIGNMENT (( #534 ) ) ;
#16486=ADVANCED_FACE ( 'NONE', ( #6025 ), #10180, .T. ) ;
#16531=VECTOR ( 'NONE', #3383, 1000.000000000000000 ) ;
#16546=VERTEX_POINT ( 'NONE', #6727 ) ;
#16592=CYLINDRICAL_SURFACE ( 'NONE', #12941, 24.99999999999999645 ) ;
#16593=VECTOR ( 'NONE', #6656, 1000.000000000000000 ) ;
#16656=SURFACE_STYLE_FILL_AREA ( #11063 ) ;
#16699=VERTEX_POINT ( 'NONE', #15209 ) ;
#16763=CARTESIAN_POINT ( 'NONE',  ( -45.00000000000000711, 171.6227766016838245, 0.000000000000000000 ) ) ;
#16795=DIRECTION ( 'NONE',  ( 1.000000000000000000, 0.000000000000000000, 0.000000000000000000 ) ) ;
#16904=CYLINDRICAL_SURFACE ( 'NONE', #6768, 19.49999999999998934 ) ;
#16913=EDGE_LOOP ( 'NONE', ( #2961, #11980, #3457, #4836 ) ) ;
#16914=CARTESIAN_POINT ( 'NONE',  ( -73.00000000000001421, 171.6227766016838245, 0.000000000000000000 ) ) ;
#16994=CARTESIAN_POINT ( 'NONE',  ( -103.0000000000000142, 171.6227766016838245, 0.000000000000000000 ) ) ;
#17015=CARTESIAN_POINT ( 'NONE',  ( -103.0000000000000142, 171.6227766016838245, 5.000000000000007994 ) ) ;
#17135=VERTEX_POINT ( 'NONE', #10136 ) ;
#17156=CARTESIAN_POINT ( 'NONE',  ( -73.00000000000001421, 171.6227766016838245, 0.000000000000000000 ) ) ;
#17228=VECTOR ( 'NONE', #3169, 1000.000000000000000 ) ;
#17232=AXIS2_PLACEMENT_3D ( 'NONE', #11417, #1873, #8850 ) ;
#17247=ORIENTED_EDGE ( 'NONE', *, *, #7335, .F. ) ;
#17326=( NAMED_UNIT ( * ) SI_UNIT ( $, .STERADIAN. ) SOLID_ANGLE_UNIT ( ) );
#17351=ADVANCED_FACE ( 'NONE', ( #8441 ), #16592, .T. ) ;
#17427=EDGE_CURVE ( 'NONE', #5867, #9898, #9286, .T. ) ;
#17505=CARTESIAN_POINT ( 'NONE',  ( -50.00000000000000000, 171.6227766016838245, -19.49999999999998224 ) ) ;
#17522=DIRECTION ( 'NONE',  ( -1.000000000000000000, 0.000000000000000000, 0.000000000000000000 ) ) ;
ENDSEC;
END-ISO-10303-21;
